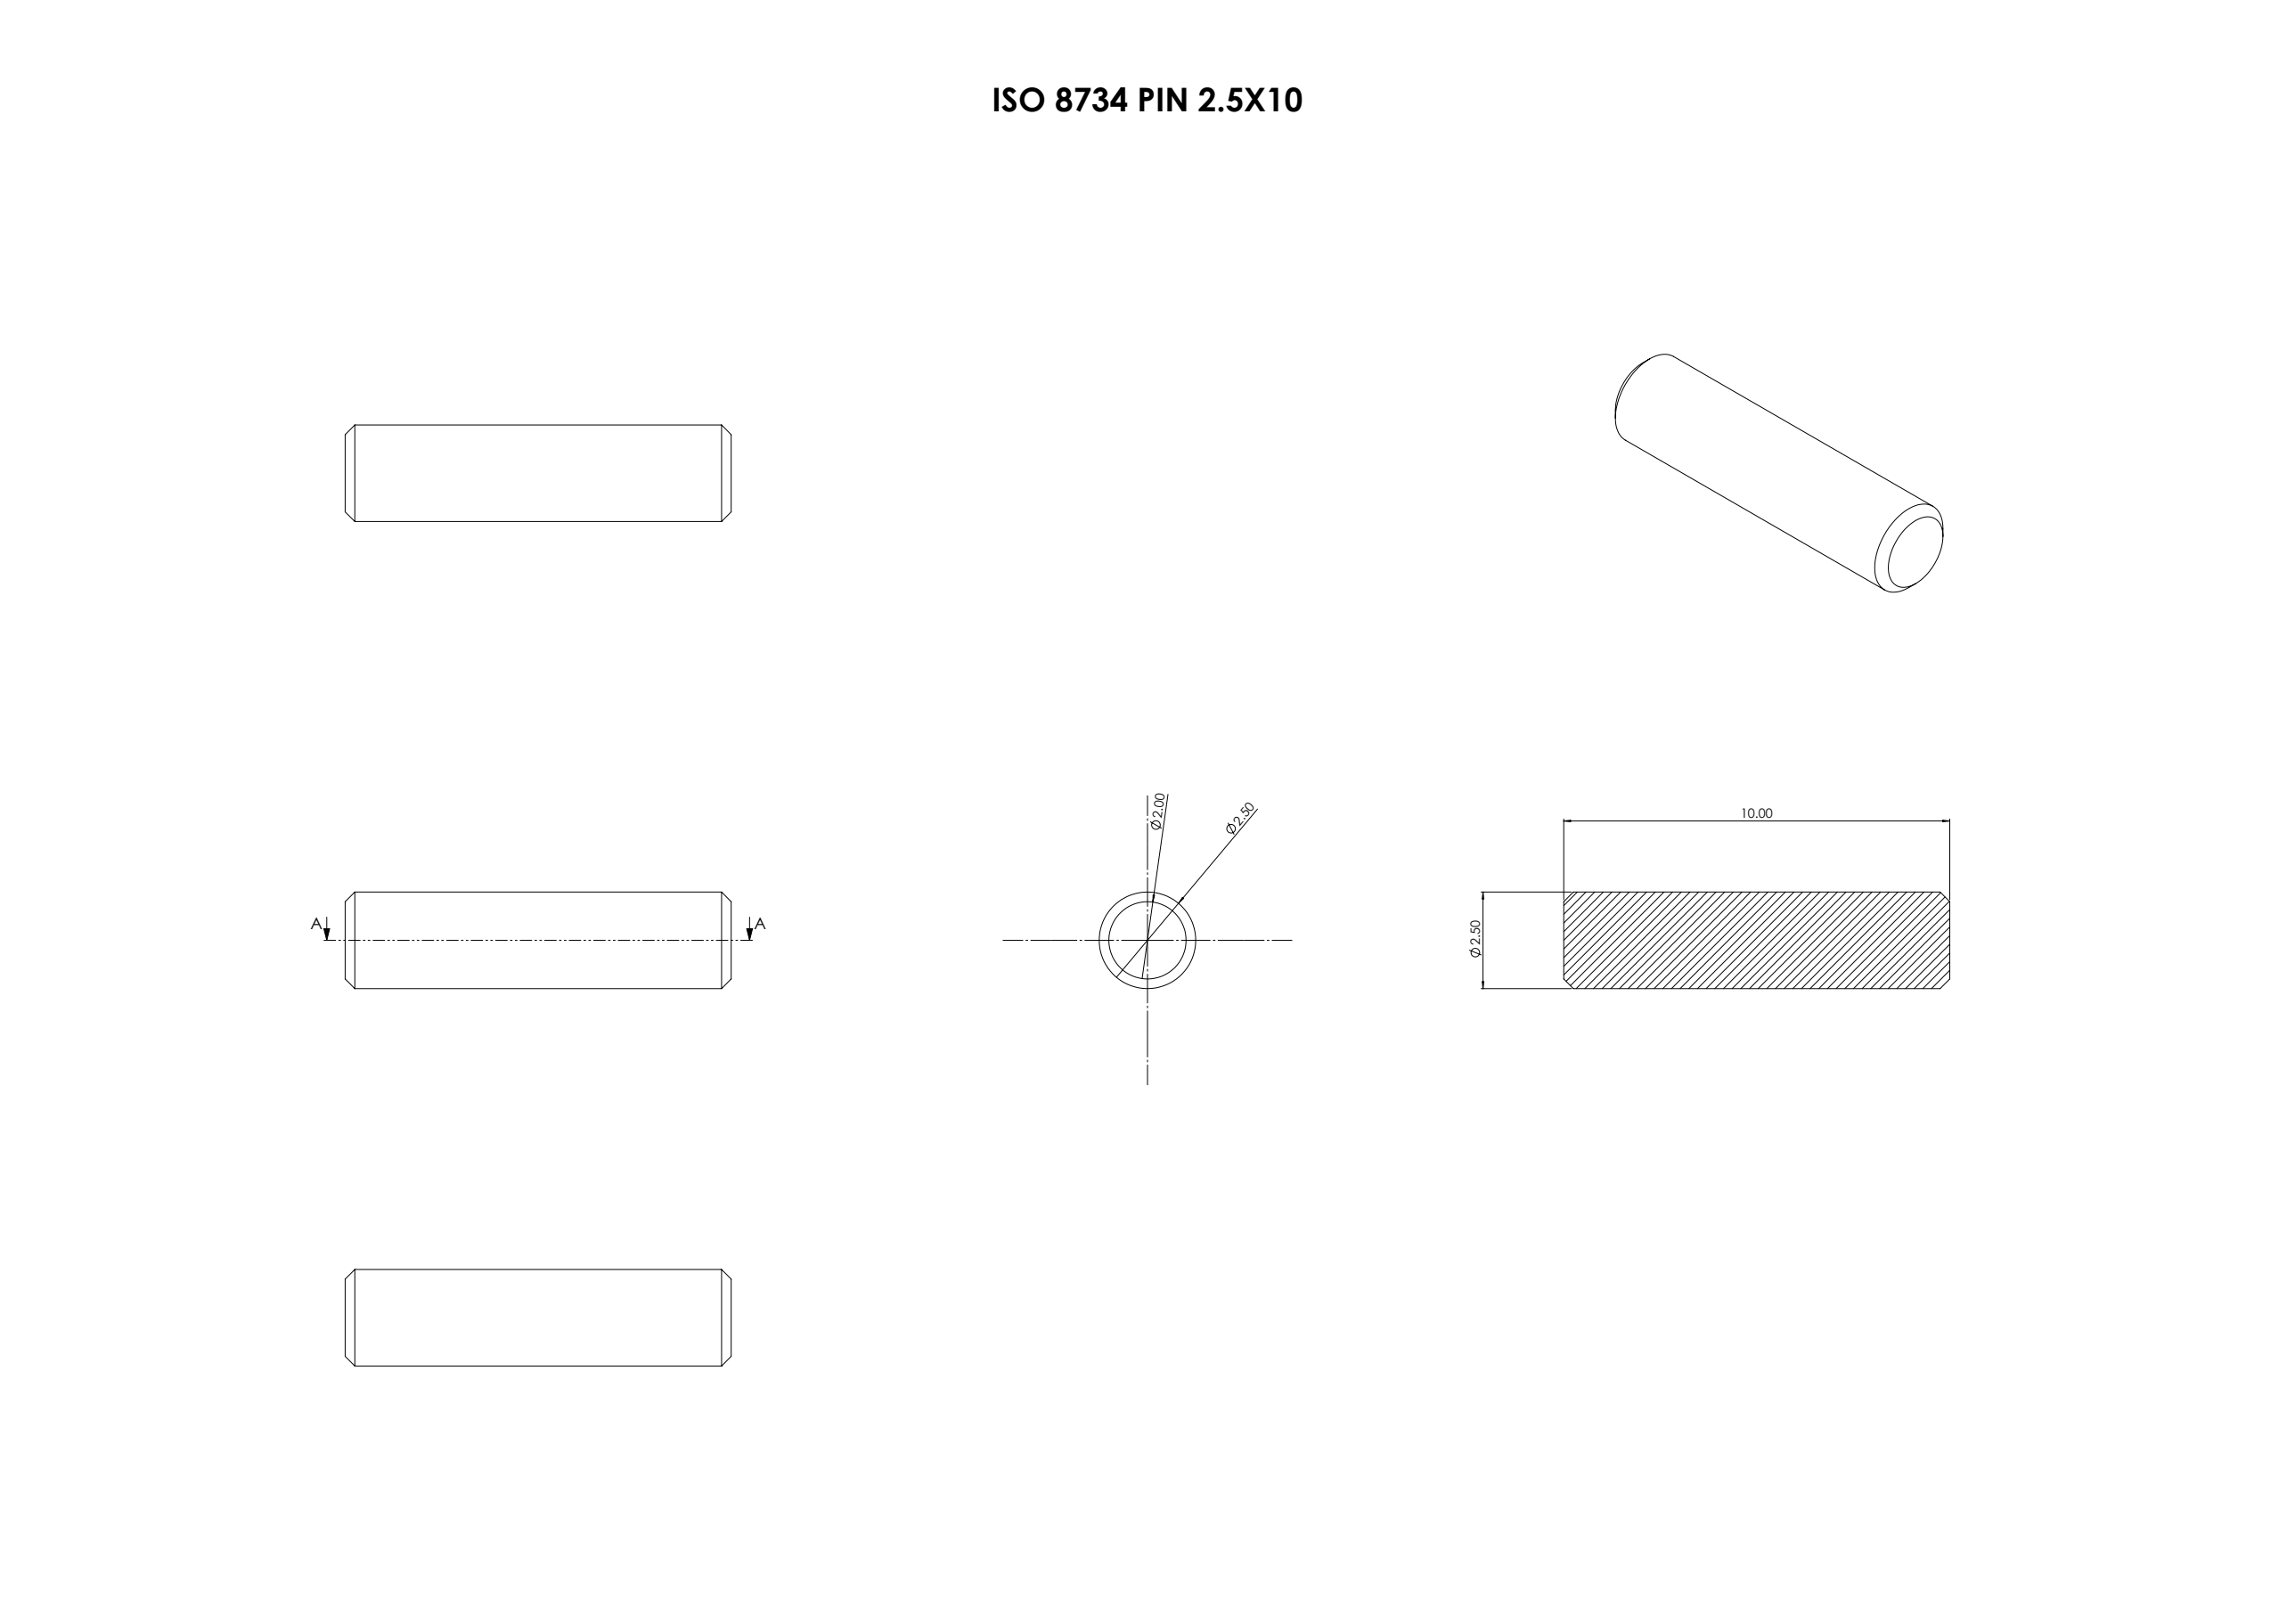
ISO-10303-21;
HEADER;
/* Generated by software containing ST-Developer
 * from STEP Tools, Inc. (www.steptools.com) 
 */

FILE_DESCRIPTION(
/* description */ (''),
/* implementation_level */ '2;1');

FILE_NAME(
/* name */ '04_ISO_8734_Pin_2.5x10.step',
/* time_stamp */ '2026-10-11T08:53:36-07:00',
/* author */ (''),
/* organization */ (''),
/* preprocessor_version */ 'ST-DEVELOPER v20.2',
/* originating_system */ 'Autodesk Translation Framework v15.15.0.0',
/* authorisation */ '');

FILE_SCHEMA (('AUTOMOTIVE_DESIGN { 1 0 10303 214 3 1 1 }'));
ENDSEC;

DATA;
#10=MECHANICAL_DESIGN_GEOMETRIC_PRESENTATION_REPRESENTATION('',(#75),#3338);
#67=SHAPE_REPRESENTATION_RELATIONSHIP('SRR','None',#3370,#71);
#71=ADVANCED_BREP_SHAPE_REPRESENTATION('',(#79),#3337);
#75=STYLED_ITEM('',(#3457),#79);
#79=MANIFOLD_SOLID_BREP('Body1',#1577);
#138=CYLINDRICAL_SURFACE('',#1800,1.25);
#189=PLANE('',#1796);
#190=PLANE('',#1804);
#278=FACE_OUTER_BOUND('',#400,.T.);
#279=FACE_OUTER_BOUND('',#401,.T.);
#280=FACE_OUTER_BOUND('',#402,.T.);
#281=FACE_OUTER_BOUND('',#403,.T.);
#282=FACE_OUTER_BOUND('',#404,.T.);
#400=EDGE_LOOP('',(#1430));
#401=EDGE_LOOP('',(#1431,#1432,#1433,#1434));
#402=EDGE_LOOP('',(#1435,#1436,#1437,#1438));
#403=EDGE_LOOP('',(#1439,#1440,#1441,#1442));
#404=EDGE_LOOP('',(#1443));
#499=LINE('',#3304,#596);
#500=LINE('',#3308,#597);
#501=LINE('',#3312,#598);
#596=VECTOR('',#2266,1.125);
#597=VECTOR('',#2271,1.25);
#598=VECTOR('',#2276,1.125);
#680=CIRCLE('',#1797,1.);
#681=CIRCLE('',#1799,1.25);
#682=CIRCLE('',#1801,1.25);
#683=CIRCLE('',#1803,1.);
#810=VERTEX_POINT('',#3299);
#811=VERTEX_POINT('',#3302);
#812=VERTEX_POINT('',#3306);
#813=VERTEX_POINT('',#3310);
#1017=EDGE_CURVE('',#810,#810,#680,.T.);
#1018=EDGE_CURVE('',#811,#811,#681,.T.);
#1019=EDGE_CURVE('',#811,#810,#499,.T.);
#1020=EDGE_CURVE('',#812,#812,#682,.T.);
#1021=EDGE_CURVE('',#812,#811,#500,.T.);
#1022=EDGE_CURVE('',#813,#813,#683,.T.);
#1023=EDGE_CURVE('',#813,#812,#501,.T.);
#1430=ORIENTED_EDGE('',*,*,#1017,.F.);
#1431=ORIENTED_EDGE('',*,*,#1018,.F.);
#1432=ORIENTED_EDGE('',*,*,#1019,.T.);
#1433=ORIENTED_EDGE('',*,*,#1017,.T.);
#1434=ORIENTED_EDGE('',*,*,#1019,.F.);
#1435=ORIENTED_EDGE('',*,*,#1020,.F.);
#1436=ORIENTED_EDGE('',*,*,#1021,.T.);
#1437=ORIENTED_EDGE('',*,*,#1018,.T.);
#1438=ORIENTED_EDGE('',*,*,#1021,.F.);
#1439=ORIENTED_EDGE('',*,*,#1022,.F.);
#1440=ORIENTED_EDGE('',*,*,#1023,.T.);
#1441=ORIENTED_EDGE('',*,*,#1020,.T.);
#1442=ORIENTED_EDGE('',*,*,#1023,.F.);
#1443=ORIENTED_EDGE('',*,*,#1022,.T.);
#1480=CONICAL_SURFACE('',#1798,1.125,0.785398163397448);
#1481=CONICAL_SURFACE('',#1802,1.125,0.785398163397448);
#1569=ADVANCED_FACE('',(#278),#189,.T.);
#1570=ADVANCED_FACE('',(#279),#1480,.T.);
#1571=ADVANCED_FACE('',(#280),#138,.T.);
#1572=ADVANCED_FACE('',(#281),#1481,.T.);
#1573=ADVANCED_FACE('',(#282),#190,.T.);
#1577=CLOSED_SHELL('',(#1569,#1570,#1571,#1572,#1573));
#1795=AXIS2_PLACEMENT_3D('',#3297,#2256,#2257);
#1796=AXIS2_PLACEMENT_3D('',#3298,#2258,#2259);
#1797=AXIS2_PLACEMENT_3D('',#3300,#2260,#2261);
#1798=AXIS2_PLACEMENT_3D('',#3301,#2262,#2263);
#1799=AXIS2_PLACEMENT_3D('',#3303,#2264,#2265);
#1800=AXIS2_PLACEMENT_3D('',#3305,#2267,#2268);
#1801=AXIS2_PLACEMENT_3D('',#3307,#2269,#2270);
#1802=AXIS2_PLACEMENT_3D('',#3309,#2272,#2273);
#1803=AXIS2_PLACEMENT_3D('',#3311,#2274,#2275);
#1804=AXIS2_PLACEMENT_3D('',#3313,#2277,#2278);
#2256=DIRECTION('axis',(0.,0.,1.));
#2257=DIRECTION('refdir',(1.,0.,0.));
#2258=DIRECTION('center_axis',(-1.,0.,0.));
#2259=DIRECTION('ref_axis',(0.,0.,1.));
#2260=DIRECTION('center_axis',(1.,0.,0.));
#2261=DIRECTION('ref_axis',(0.,0.,-1.));
#2262=DIRECTION('center_axis',(1.,0.,0.));
#2263=DIRECTION('ref_axis',(0.,1.,0.));
#2264=DIRECTION('center_axis',(1.,0.,0.));
#2265=DIRECTION('ref_axis',(0.,0.,-1.));
#2266=DIRECTION('',(-0.707106781186548,0.707106781186547,8.65956056235493E-17));
#2267=DIRECTION('center_axis',(1.,0.,0.));
#2268=DIRECTION('ref_axis',(0.,1.,0.));
#2269=DIRECTION('center_axis',(1.,0.,0.));
#2270=DIRECTION('ref_axis',(0.,0.,-1.));
#2271=DIRECTION('',(-1.,0.,0.));
#2272=DIRECTION('center_axis',(-1.,0.,0.));
#2273=DIRECTION('ref_axis',(0.,1.,0.));
#2274=DIRECTION('center_axis',(1.,0.,0.));
#2275=DIRECTION('ref_axis',(0.,0.,-1.));
#2276=DIRECTION('',(-0.707106781186548,-0.707106781186547,-8.65956056235493E-17));
#2277=DIRECTION('center_axis',(1.,0.,0.));
#2278=DIRECTION('ref_axis',(0.,0.,-1.));
#3297=CARTESIAN_POINT('',(0.,0.,0.));
#3298=CARTESIAN_POINT('Origin',(0.,1.,0.));
#3299=CARTESIAN_POINT('',(-2.25514051876985E-16,-1.,-1.22464679914735E-16));
#3300=CARTESIAN_POINT('Origin',(0.,0.,0.));
#3301=CARTESIAN_POINT('Origin',(0.125,0.,0.));
#3302=CARTESIAN_POINT('',(0.25,-1.25,-1.53080849893419E-16));
#3303=CARTESIAN_POINT('Origin',(0.25,0.,0.));
#3304=CARTESIAN_POINT('',(0.125,-1.125,-1.37772764904077E-16));
#3305=CARTESIAN_POINT('Origin',(5.,0.,0.));
#3306=CARTESIAN_POINT('',(9.75,-1.25,-1.53080849893419E-16));
#3307=CARTESIAN_POINT('Origin',(9.75,0.,0.));
#3308=CARTESIAN_POINT('',(5.,-1.25,-1.53080849893419E-16));
#3309=CARTESIAN_POINT('Origin',(9.875,0.,0.));
#3310=CARTESIAN_POINT('',(10.,-1.,-1.22464679914735E-16));
#3311=CARTESIAN_POINT('Origin',(10.,0.,0.));
#3312=CARTESIAN_POINT('',(9.875,-1.125,-1.37772764904077E-16));
#3313=CARTESIAN_POINT('Origin',(10.,0.,0.));
#3331=UNCERTAINTY_MEASURE_WITH_UNIT(LENGTH_MEASURE(0.01),#3339,
'DISTANCE_ACCURACY_VALUE',
'Maximum model space distance between geometric entities at asserted c
onnectivities');
#3332=UNCERTAINTY_MEASURE_WITH_UNIT(LENGTH_MEASURE(0.01),#3339,
'DISTANCE_ACCURACY_VALUE',
'Maximum model space distance between geometric entities at asserted c
onnectivities');
#3337=(
GEOMETRIC_REPRESENTATION_CONTEXT(3)
GLOBAL_UNCERTAINTY_ASSIGNED_CONTEXT((#3331))
GLOBAL_UNIT_ASSIGNED_CONTEXT((#3339,#3341,#3342))
REPRESENTATION_CONTEXT('','3D')
);
#3338=(
GEOMETRIC_REPRESENTATION_CONTEXT(3)
GLOBAL_UNCERTAINTY_ASSIGNED_CONTEXT((#3332))
GLOBAL_UNIT_ASSIGNED_CONTEXT((#3339,#3341,#3342))
REPRESENTATION_CONTEXT('','3D')
);
#3339=(
LENGTH_UNIT()
NAMED_UNIT(*)
SI_UNIT(.MILLI.,.METRE.)
);
#3341=(
NAMED_UNIT(*)
PLANE_ANGLE_UNIT()
SI_UNIT($,.RADIAN.)
);
#3342=(
NAMED_UNIT(*)
SI_UNIT($,.STERADIAN.)
SOLID_ANGLE_UNIT()
);
#3347=SHAPE_DEFINITION_REPRESENTATION(#3352,#3370);
#3352=PRODUCT_DEFINITION_SHAPE('',$,#3376);
#3370=SHAPE_REPRESENTATION('',(#1795),#3337);
#3371=PRODUCT_DEFINITION_CONTEXT('part definition',#3388,'design');
#3376=PRODUCT_DEFINITION('2026-10-11-08-53-16-748',
'04_ISO_8734_Pin_2.5x10',#3381,#3371);
#3381=PRODUCT_DEFINITION_FORMATION('',$,#3394);
#3388=APPLICATION_CONTEXT(
'Core Data for Automotive Mechanical Design Process');
#3389=PRODUCT_CONTEXT('part definition',#3388,'mechanical');
#3394=PRODUCT('2026-10-11-08-53-16-748','04_ISO_8734_Pin_2.5x10',$,(#3389));
#3451=COLOUR_RGB('Grey',0.48,0.52,0.57);
#3452=FILL_AREA_STYLE_COLOUR('',#3451);
#3453=FILL_AREA_STYLE('',(#3452));
#3454=SURFACE_STYLE_FILL_AREA(#3453);
#3455=SURFACE_SIDE_STYLE('',(#3454));
#3456=SURFACE_STYLE_USAGE(.BOTH.,#3455);
#3457=PRESENTATION_STYLE_ASSIGNMENT((#3456));
ENDSEC;
END-ISO-10303-21;
